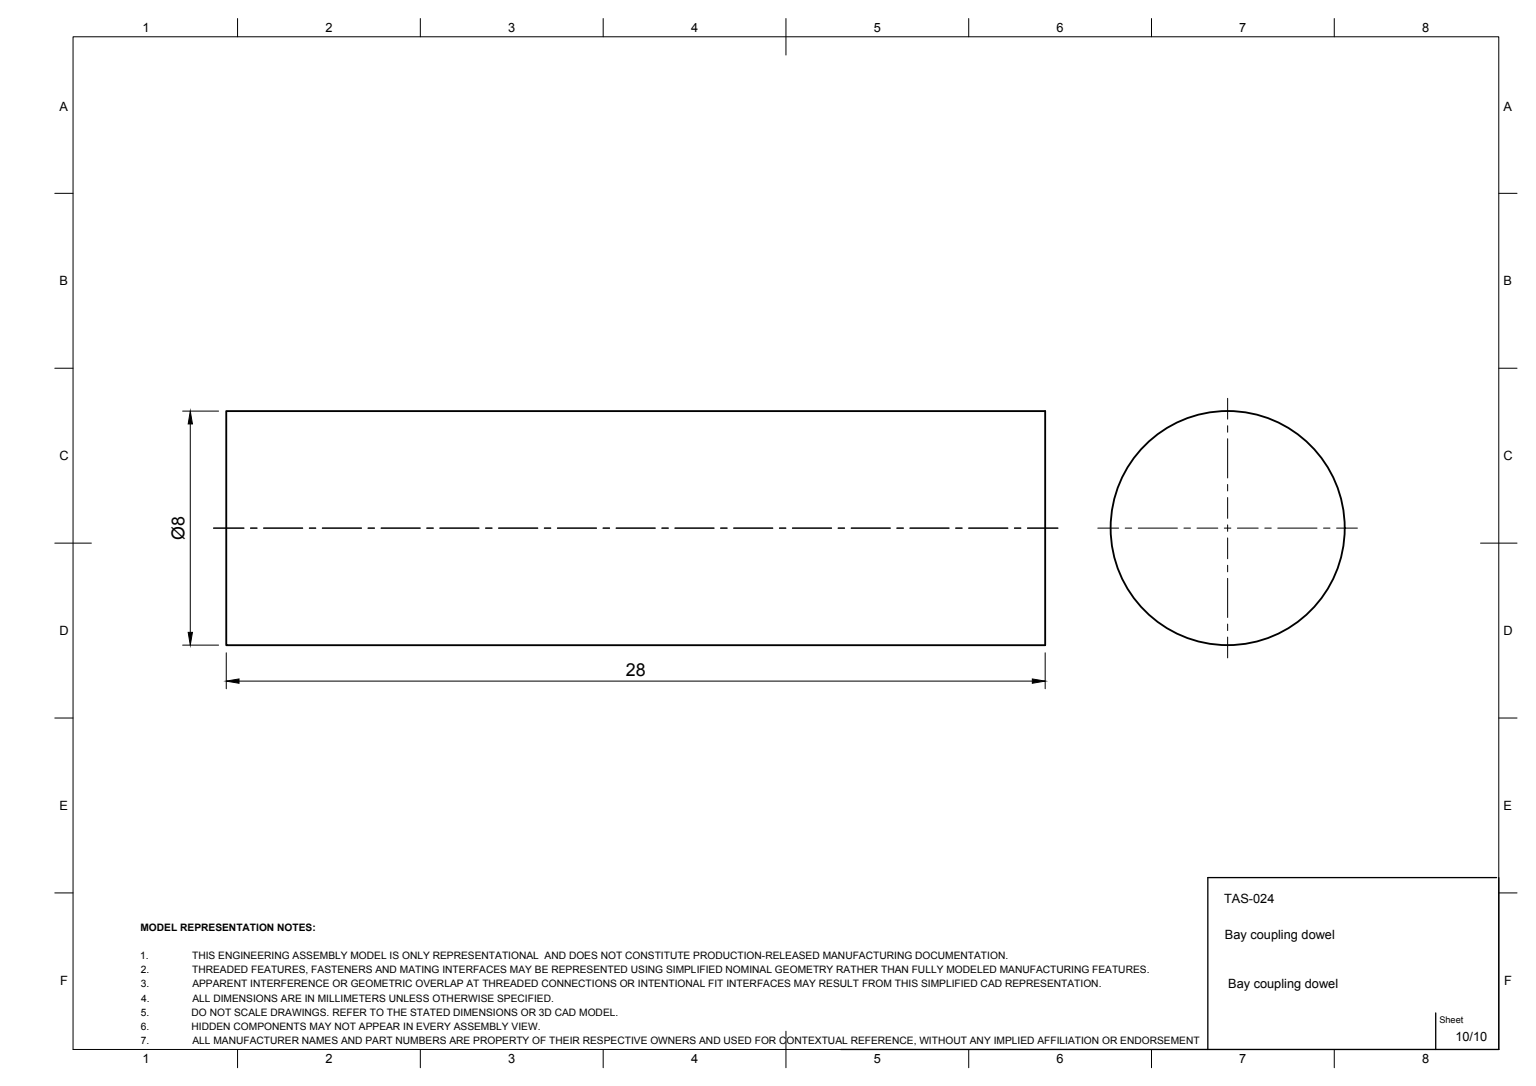
ISO-10303-21;
HEADER;
/* Generated by software containing ST-Developer
 * from STEP Tools, Inc. (www.steptools.com) 
 */

FILE_DESCRIPTION(
/* description */ (''),
/* implementation_level */ '2;1');

FILE_NAME(
/* name */ 'Bay coupling dowel.step',
/* time_stamp */ '2026-11-15T17:53:25-08:00',
/* author */ (''),
/* organization */ (''),
/* preprocessor_version */ 'ST-DEVELOPER v20.2',
/* originating_system */ 'Autodesk Translation Framework v15.17.0.0',
/* authorisation */ '');

FILE_SCHEMA (('AUTOMOTIVE_DESIGN { 1 0 10303 214 3 1 1 }'));
ENDSEC;

DATA;
#10=MECHANICAL_DESIGN_GEOMETRIC_PRESENTATION_REPRESENTATION('',(#138),#2673);
#122=SHAPE_REPRESENTATION_RELATIONSHIP('SRR','None',#2730,#130);
#130=ADVANCED_BREP_SHAPE_REPRESENTATION('',(#146),#2672);
#138=STYLED_ITEM('',(#2779),#146);
#146=MANIFOLD_SOLID_BREP('Body1',#1524);
#231=PLANE('',#1742);
#232=PLANE('',#1743);
#319=FACE_OUTER_BOUND('',#421,.T.);
#320=FACE_OUTER_BOUND('',#422,.T.);
#321=FACE_OUTER_BOUND('',#423,.T.);
#421=EDGE_LOOP('',(#1406,#1407,#1408,#1409));
#422=EDGE_LOOP('',(#1410));
#423=EDGE_LOOP('',(#1411));
#571=LINE('',#2624,#719);
#719=VECTOR('',#2171,0.4);
#750=CIRCLE('',#1740,0.4);
#751=CIRCLE('',#1741,0.4);
#870=VERTEX_POINT('',#2621);
#871=VERTEX_POINT('',#2623);
#1049=EDGE_CURVE('',#870,#870,#750,.T.);
#1050=EDGE_CURVE('',#870,#871,#571,.T.);
#1051=EDGE_CURVE('',#871,#871,#751,.T.);
#1406=ORIENTED_EDGE('',*,*,#1049,.F.);
#1407=ORIENTED_EDGE('',*,*,#1050,.T.);
#1408=ORIENTED_EDGE('',*,*,#1051,.T.);
#1409=ORIENTED_EDGE('',*,*,#1050,.F.);
#1410=ORIENTED_EDGE('',*,*,#1049,.T.);
#1411=ORIENTED_EDGE('',*,*,#1051,.F.);
#1427=CYLINDRICAL_SURFACE('',#1739,0.4);
#1514=ADVANCED_FACE('',(#319),#1427,.T.);
#1515=ADVANCED_FACE('',(#320),#231,.T.);
#1516=ADVANCED_FACE('',(#321),#232,.F.);
#1524=CLOSED_SHELL('',(#1514,#1515,#1516));
#1738=AXIS2_PLACEMENT_3D('',#2619,#2165,#2166);
#1739=AXIS2_PLACEMENT_3D('',#2620,#2167,#2168);
#1740=AXIS2_PLACEMENT_3D('',#2622,#2169,#2170);
#1741=AXIS2_PLACEMENT_3D('',#2625,#2172,#2173);
#1742=AXIS2_PLACEMENT_3D('',#2626,#2174,#2175);
#1743=AXIS2_PLACEMENT_3D('',#2627,#2176,#2177);
#2165=DIRECTION('axis',(0.,0.,1.));
#2166=DIRECTION('refdir',(1.,0.,0.));
#2167=DIRECTION('center_axis',(0.,0.,1.));
#2168=DIRECTION('ref_axis',(1.,0.,0.));
#2169=DIRECTION('center_axis',(0.,0.,1.));
#2170=DIRECTION('ref_axis',(1.,0.,0.));
#2171=DIRECTION('',(0.,0.,-1.));
#2172=DIRECTION('center_axis',(0.,0.,1.));
#2173=DIRECTION('ref_axis',(1.,0.,0.));
#2174=DIRECTION('center_axis',(0.,0.,1.));
#2175=DIRECTION('ref_axis',(1.,0.,0.));
#2176=DIRECTION('center_axis',(0.,0.,1.));
#2177=DIRECTION('ref_axis',(1.,0.,0.));
#2619=CARTESIAN_POINT('',(0.,0.,0.));
#2620=CARTESIAN_POINT('Origin',(0.,0.,0.));
#2621=CARTESIAN_POINT('',(-0.4,-4.89858719658941E-17,2.8));
#2622=CARTESIAN_POINT('Origin',(0.,0.,2.8));
#2623=CARTESIAN_POINT('',(-0.4,-4.89858719658941E-17,0.));
#2624=CARTESIAN_POINT('',(-0.4,-4.89858719658941E-17,0.));
#2625=CARTESIAN_POINT('Origin',(0.,0.,0.));
#2626=CARTESIAN_POINT('Origin',(0.,0.,2.8));
#2627=CARTESIAN_POINT('Origin',(0.,0.,0.));
#2662=UNCERTAINTY_MEASURE_WITH_UNIT(LENGTH_MEASURE(0.001),#2674,
'DISTANCE_ACCURACY_VALUE',
'Maximum model space distance between geometric entities at asserted c
onnectivities');
#2663=UNCERTAINTY_MEASURE_WITH_UNIT(LENGTH_MEASURE(0.001),#2674,
'DISTANCE_ACCURACY_VALUE',
'Maximum model space distance between geometric entities at asserted c
onnectivities');
#2672=(
GEOMETRIC_REPRESENTATION_CONTEXT(3)
GLOBAL_UNCERTAINTY_ASSIGNED_CONTEXT((#2662))
GLOBAL_UNIT_ASSIGNED_CONTEXT((#2674,#2676,#2677))
REPRESENTATION_CONTEXT('','3D')
);
#2673=(
GEOMETRIC_REPRESENTATION_CONTEXT(3)
GLOBAL_UNCERTAINTY_ASSIGNED_CONTEXT((#2663))
GLOBAL_UNIT_ASSIGNED_CONTEXT((#2674,#2676,#2677))
REPRESENTATION_CONTEXT('','3D')
);
#2674=(
LENGTH_UNIT()
NAMED_UNIT(*)
SI_UNIT(.CENTI.,.METRE.)
);
#2676=(
NAMED_UNIT(*)
PLANE_ANGLE_UNIT()
SI_UNIT($,.RADIAN.)
);
#2677=(
NAMED_UNIT(*)
SI_UNIT($,.STERADIAN.)
SOLID_ANGLE_UNIT()
);
#2686=SHAPE_DEFINITION_REPRESENTATION(#2695,#2730);
#2695=PRODUCT_DEFINITION_SHAPE('',$,#2740);
#2730=SHAPE_REPRESENTATION('',(#1738),#2672);
#2731=PRODUCT_DEFINITION_CONTEXT('part definition',#2760,'design');
#2740=PRODUCT_DEFINITION('Bay coupling dowel','Bay coupling dowel',#2749,
#2731);
#2749=PRODUCT_DEFINITION_FORMATION('',$,#2770);
#2760=APPLICATION_CONTEXT(
'Core Data for Automotive Mechanical Design Process');
#2761=PRODUCT_CONTEXT('part definition',#2760,'mechanical');
#2770=PRODUCT('Bay coupling dowel','Bay coupling dowel',$,(#2761));
#2779=PRESENTATION_STYLE_ASSIGNMENT((#2788));
#2788=SURFACE_STYLE_USAGE(.BOTH.,#2797);
#2797=SURFACE_SIDE_STYLE('',(#2806));
#2806=SURFACE_STYLE_FILL_AREA(#2815);
#2815=FILL_AREA_STYLE('Bay coupling dowel finish',(#2824));
#2824=FILL_AREA_STYLE_COLOUR('Bay coupling dowel finish',#2833);
#2833=COLOUR_RGB('Bay coupling dowel finish',0.43921568627451,0.47843137254902,
0.52156862745098);
ENDSEC;
END-ISO-10303-21;
